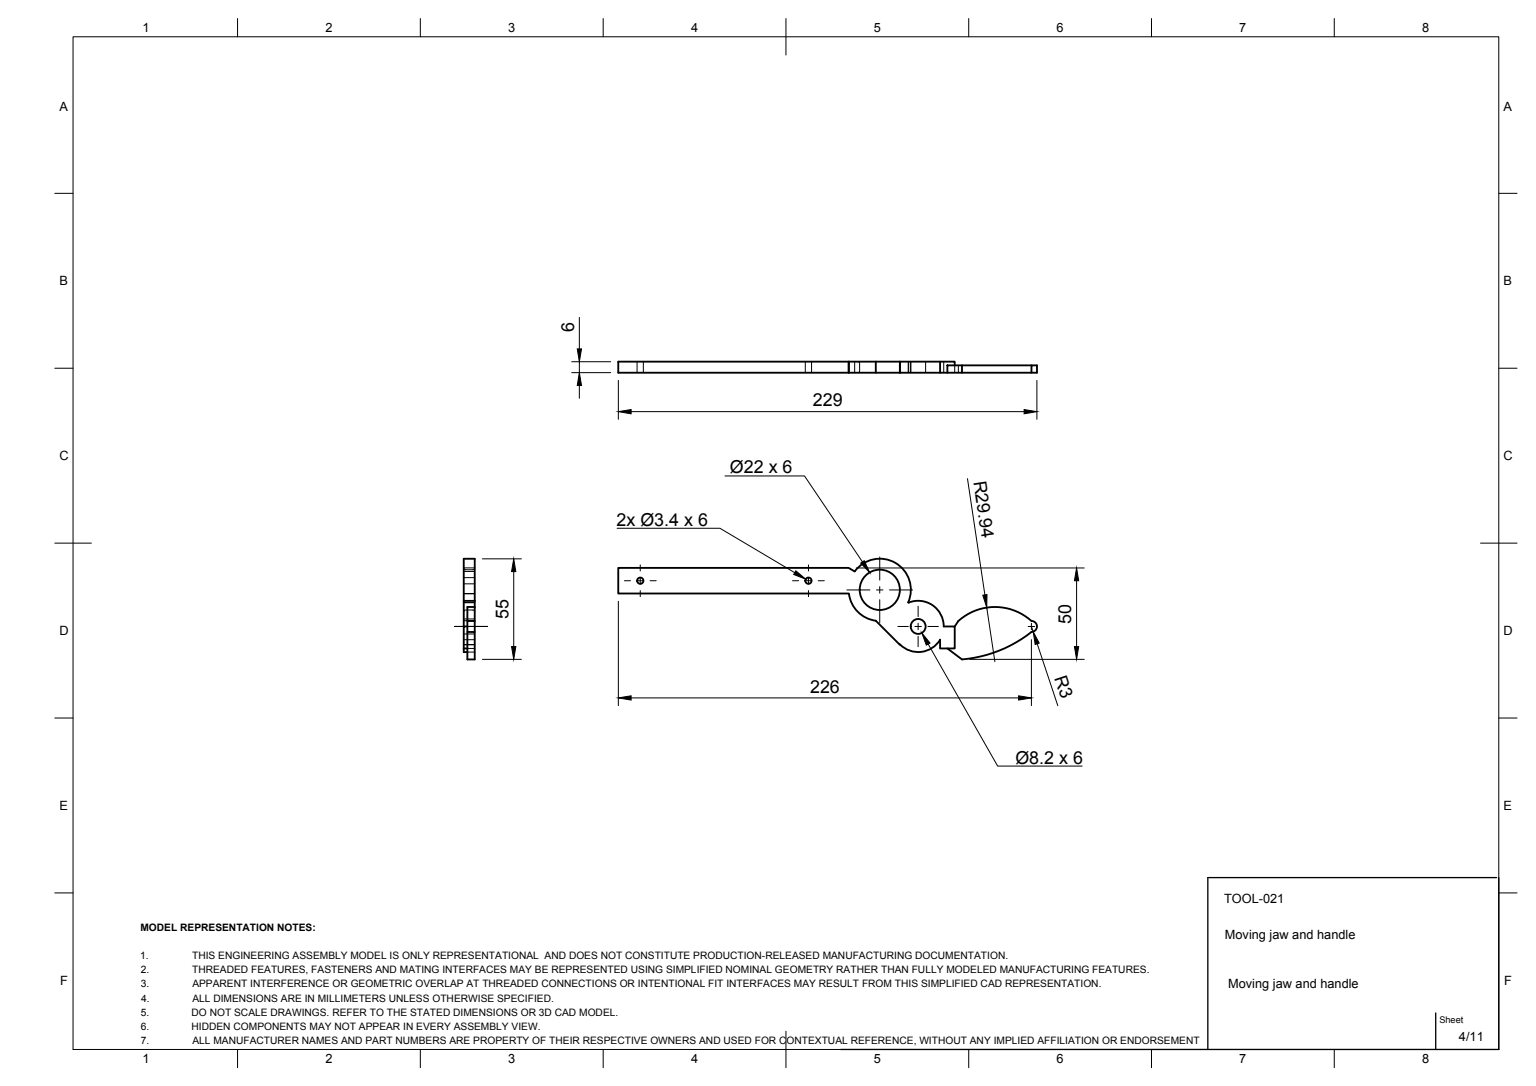
ISO-10303-21;
HEADER;
/* Generated by software containing ST-Developer
 * from STEP Tools, Inc. (www.steptools.com) 
 */

FILE_DESCRIPTION(
/* description */ (''),
/* implementation_level */ '2;1');

FILE_NAME(
/* name */ 'Moving jaw and handle.step',
/* time_stamp */ '2026-11-10T09:05:57-08:00',
/* author */ (''),
/* organization */ (''),
/* preprocessor_version */ 'ST-DEVELOPER v20.2',
/* originating_system */ 'Autodesk Translation Framework v15.17.0.0',
/* authorisation */ '');

FILE_SCHEMA (('AUTOMOTIVE_DESIGN { 1 0 10303 214 3 1 1 }'));
ENDSEC;

DATA;
#10=MECHANICAL_DESIGN_GEOMETRIC_PRESENTATION_REPRESENTATION('',(#566),#19618);
#546=SHAPE_REPRESENTATION_RELATIONSHIP('SRR','None',#19665,#556);
#556=ADVANCED_BREP_SHAPE_REPRESENTATION('',(#576),#19608);
#566=STYLED_ITEM('',(#19728),#576);
#576=MANIFOLD_SOLID_BREP('Body1',#7104);
#587=TOROIDAL_SURFACE('',#7321,1.2,0.1);
#588=TOROIDAL_SURFACE('',#7331,1.2,0.1);
#597=FACE_BOUND('',#1280,.T.);
#598=FACE_BOUND('',#1281,.T.);
#599=FACE_BOUND('',#1282,.T.);
#600=FACE_BOUND('',#1283,.T.);
#601=FACE_BOUND('',#1287,.T.);
#602=FACE_BOUND('',#1288,.T.);
#603=FACE_BOUND('',#1289,.T.);
#604=FACE_BOUND('',#1290,.T.);
#681=PLANE('',#7295);
#682=PLANE('',#7296);
#683=PLANE('',#7306);
#684=PLANE('',#7307);
#685=PLANE('',#7308);
#686=PLANE('',#7309);
#687=PLANE('',#7310);
#688=PLANE('',#7317);
#689=PLANE('',#7328);
#690=PLANE('',#7335);
#691=PLANE('',#7336);
#692=PLANE('',#7337);
#693=PLANE('',#7338);
#694=PLANE('',#7339);
#695=PLANE('',#7340);
#696=PLANE('',#7341);
#697=PLANE('',#7342);
#853=FACE_OUTER_BOUND('',#1264,.T.);
#854=FACE_OUTER_BOUND('',#1265,.T.);
#855=FACE_OUTER_BOUND('',#1266,.T.);
#856=FACE_OUTER_BOUND('',#1267,.T.);
#857=FACE_OUTER_BOUND('',#1268,.T.);
#858=FACE_OUTER_BOUND('',#1269,.T.);
#859=FACE_OUTER_BOUND('',#1270,.T.);
#860=FACE_OUTER_BOUND('',#1271,.T.);
#861=FACE_OUTER_BOUND('',#1272,.T.);
#862=FACE_OUTER_BOUND('',#1273,.T.);
#863=FACE_OUTER_BOUND('',#1274,.T.);
#864=FACE_OUTER_BOUND('',#1275,.T.);
#865=FACE_OUTER_BOUND('',#1276,.T.);
#866=FACE_OUTER_BOUND('',#1277,.T.);
#867=FACE_OUTER_BOUND('',#1278,.T.);
#868=FACE_OUTER_BOUND('',#1279,.T.);
#869=FACE_OUTER_BOUND('',#1284,.T.);
#870=FACE_OUTER_BOUND('',#1285,.T.);
#871=FACE_OUTER_BOUND('',#1286,.T.);
#872=FACE_OUTER_BOUND('',#1291,.T.);
#873=FACE_OUTER_BOUND('',#1292,.T.);
#874=FACE_OUTER_BOUND('',#1293,.T.);
#875=FACE_OUTER_BOUND('',#1294,.T.);
#876=FACE_OUTER_BOUND('',#1295,.T.);
#877=FACE_OUTER_BOUND('',#1296,.T.);
#878=FACE_OUTER_BOUND('',#1297,.T.);
#879=FACE_OUTER_BOUND('',#1298,.T.);
#880=FACE_OUTER_BOUND('',#1299,.T.);
#881=FACE_OUTER_BOUND('',#1300,.T.);
#882=FACE_OUTER_BOUND('',#1301,.T.);
#1264=EDGE_LOOP('',(#4678,#4679,#4680,#4681));
#1265=EDGE_LOOP('',(#4682,#4683,#4684,#4685));
#1266=EDGE_LOOP('',(#4686,#4687,#4688,#4689));
#1267=EDGE_LOOP('',(#4690,#4691,#4692,#4693));
#1268=EDGE_LOOP('',(#4694,#4695,#4696,#4697));
#1269=EDGE_LOOP('',(#4698,#4699,#4700,#4701));
#1270=EDGE_LOOP('',(#4702,#4703,#4704,#4705));
#1271=EDGE_LOOP('',(#4706,#4707,#4708,#4709));
#1272=EDGE_LOOP('',(#4710,#4711,#4712,#4713,#4714,#4715,#4716));
#1273=EDGE_LOOP('',(#4717,#4718,#4719,#4720,#4721,#4722));
#1274=EDGE_LOOP('',(#4723,#4724,#4725,#4726));
#1275=EDGE_LOOP('',(#4727,#4728,#4729,#4730,#4731));
#1276=EDGE_LOOP('',(#4732,#4733,#4734,#4735));
#1277=EDGE_LOOP('',(#4736,#4737,#4738,#4739));
#1278=EDGE_LOOP('',(#4740,#4741,#4742,#4743));
#1279=EDGE_LOOP('',(#4744,#4745,#4746,#4747,#4748,#4749,#4750,#4751,#4752,
#4753,#4754,#4755,#4756,#4757,#4758,#4759));
#1280=EDGE_LOOP('',(#4760));
#1281=EDGE_LOOP('',(#4761));
#1282=EDGE_LOOP('',(#4762));
#1283=EDGE_LOOP('',(#4763));
#1284=EDGE_LOOP('',(#4764,#4765,#4766,#4767));
#1285=EDGE_LOOP('',(#4768,#4769,#4770,#4771,#4772));
#1286=EDGE_LOOP('',(#4773,#4774,#4775,#4776,#4777,#4778,#4779,#4780,#4781,
#4782,#4783,#4784,#4785,#4786,#4787,#4788,#4789,#4790,#4791,#4792));
#1287=EDGE_LOOP('',(#4793));
#1288=EDGE_LOOP('',(#4794));
#1289=EDGE_LOOP('',(#4795));
#1290=EDGE_LOOP('',(#4796));
#1291=EDGE_LOOP('',(#4797,#4798,#4799,#4800,#4801));
#1292=EDGE_LOOP('',(#4802,#4803,#4804,#4805));
#1293=EDGE_LOOP('',(#4806,#4807,#4808,#4809));
#1294=EDGE_LOOP('',(#4810,#4811,#4812,#4813));
#1295=EDGE_LOOP('',(#4814,#4815,#4816,#4817));
#1296=EDGE_LOOP('',(#4818,#4819,#4820,#4821));
#1297=EDGE_LOOP('',(#4822,#4823,#4824,#4825));
#1298=EDGE_LOOP('',(#4826,#4827,#4828,#4829));
#1299=EDGE_LOOP('',(#4830,#4831,#4832,#4833));
#1300=EDGE_LOOP('',(#4834,#4835,#4836,#4837));
#1301=EDGE_LOOP('',(#4838,#4839,#4840,#4841));
#1758=LINE('',#9501,#2217);
#1759=LINE('',#9507,#2218);
#1760=LINE('',#9513,#2219);
#1761=LINE('',#9518,#2220);
#1762=LINE('',#9520,#2221);
#1763=LINE('',#9522,#2222);
#1764=LINE('',#9523,#2223);
#1765=LINE('',#9527,#2224);
#1766=LINE('',#9529,#2225);
#1767=LINE('',#9531,#2226);
#1768=LINE('',#9532,#2227);
#1769=LINE('',#9538,#2228);
#1770=LINE('',#9544,#2229);
#1771=LINE('',#9550,#2230);
#1772=LINE('',#9551,#2231);
#1773=LINE('',#9554,#2232);
#1774=LINE('',#9556,#2233);
#1775=LINE('',#9558,#2234);
#1776=LINE('',#9559,#2235);
#1777=LINE('',#9562,#2236);
#1778=LINE('',#9563,#2237);
#1779=LINE('',#9567,#2238);
#1780=LINE('',#9568,#2239);
#1781=LINE('',#9569,#2240);
#1782=LINE('',#9573,#2241);
#1783=LINE('',#9574,#2242);
#1784=LINE('',#9575,#2243);
#1785=LINE('',#9580,#2244);
#1786=LINE('',#9586,#2245);
#1787=LINE('',#9590,#2246);
#1788=LINE('',#9594,#2247);
#1789=LINE('',#9596,#2248);
#1790=LINE('',#9598,#2249);
#1791=LINE('',#9600,#2250);
#1792=LINE('',#9602,#2251);
#1793=LINE('',#9606,#2252);
#1794=LINE('',#9607,#2253);
#1795=LINE('',#9621,#2254);
#1796=LINE('',#9624,#2255);
#1797=LINE('',#9626,#2256);
#1798=LINE('',#9630,#2257);
#1799=LINE('',#9632,#2258);
#1800=LINE('',#9634,#2259);
#1801=LINE('',#9636,#2260);
#1802=LINE('',#9638,#2261);
#1803=LINE('',#9641,#2262);
#1804=LINE('',#9645,#2263);
#1805=LINE('',#9646,#2264);
#1806=LINE('',#9648,#2265);
#1807=LINE('',#9649,#2266);
#1808=LINE('',#9651,#2267);
#1809=LINE('',#9653,#2268);
#1810=LINE('',#9656,#2269);
#1811=LINE('',#9659,#2270);
#1812=LINE('',#9661,#2271);
#2217=VECTOR('',#7957,0.17);
#2218=VECTOR('',#7964,0.17);
#2219=VECTOR('',#7971,0.41);
#2220=VECTOR('',#7976,1.);
#2221=VECTOR('',#7977,1.);
#2222=VECTOR('',#7978,1.);
#2223=VECTOR('',#7979,1.);
#2224=VECTOR('',#7982,1.);
#2225=VECTOR('',#7983,1.);
#2226=VECTOR('',#7984,1.);
#2227=VECTOR('',#7985,1.);
#2228=VECTOR('',#7992,1.);
#2229=VECTOR('',#7999,1.);
#2230=VECTOR('',#8008,1.);
#2231=VECTOR('',#8009,1.);
#2232=VECTOR('',#8012,1.);
#2233=VECTOR('',#8013,1.);
#2234=VECTOR('',#8014,1.);
#2235=VECTOR('',#8015,1.);
#2236=VECTOR('',#8018,1.);
#2237=VECTOR('',#8019,1.);
#2238=VECTOR('',#8022,1.);
#2239=VECTOR('',#8023,1.);
#2240=VECTOR('',#8024,1.);
#2241=VECTOR('',#8027,1.);
#2242=VECTOR('',#8028,1.);
#2243=VECTOR('',#8029,1.);
#2244=VECTOR('',#8034,1.);
#2245=VECTOR('',#8041,1.);
#2246=VECTOR('',#8046,1.);
#2247=VECTOR('',#8049,1.);
#2248=VECTOR('',#8050,1.);
#2249=VECTOR('',#8051,1.);
#2250=VECTOR('',#8052,1.);
#2251=VECTOR('',#8053,1.);
#2252=VECTOR('',#8056,1.);
#2253=VECTOR('',#8057,1.);
#2254=VECTOR('',#8074,1.1);
#2255=VECTOR('',#8077,1.);
#2256=VECTOR('',#8078,1.);
#2257=VECTOR('',#8081,1.);
#2258=VECTOR('',#8082,1.);
#2259=VECTOR('',#8083,1.);
#2260=VECTOR('',#8084,1.);
#2261=VECTOR('',#8085,1.);
#2262=VECTOR('',#8088,1.);
#2263=VECTOR('',#8095,1.);
#2264=VECTOR('',#8096,1.);
#2265=VECTOR('',#8099,1.);
#2266=VECTOR('',#8100,1.);
#2267=VECTOR('',#8103,1.);
#2268=VECTOR('',#8106,1.);
#2269=VECTOR('',#8111,1.);
#2270=VECTOR('',#8116,1.);
#2271=VECTOR('',#8119,1.);
#2643=CIRCLE('',#7287,0.17);
#2644=CIRCLE('',#7288,0.17);
#2645=CIRCLE('',#7290,0.17);
#2646=CIRCLE('',#7291,0.17);
#2647=CIRCLE('',#7293,0.41);
#2648=CIRCLE('',#7294,0.41);
#2649=CIRCLE('',#7298,2.9940843367589);
#2650=CIRCLE('',#7299,2.9940843367589);
#2651=CIRCLE('',#7301,0.3);
#2652=CIRCLE('',#7302,0.3);
#2653=CIRCLE('',#7304,7.11398555645532);
#2654=CIRCLE('',#7305,7.11398555645532);
#2655=CIRCLE('',#7312,1.4);
#2656=CIRCLE('',#7313,1.4);
#2657=CIRCLE('',#7315,1.4);
#2658=CIRCLE('',#7316,1.4);
#2659=CIRCLE('',#7318,1.7);
#2660=CIRCLE('',#7319,1.7);
#2661=CIRCLE('',#7320,1.2);
#2662=CIRCLE('',#7322,1.2);
#2663=CIRCLE('',#7323,0.1);
#2664=CIRCLE('',#7324,1.1);
#2665=CIRCLE('',#7326,1.1);
#2666=CIRCLE('',#7327,1.1);
#2667=CIRCLE('',#7329,1.7);
#2668=CIRCLE('',#7330,1.7);
#2669=CIRCLE('',#7332,0.1);
#2867=VERTEX_POINT('',#9498);
#2868=VERTEX_POINT('',#9500);
#2869=VERTEX_POINT('',#9504);
#2870=VERTEX_POINT('',#9506);
#2871=VERTEX_POINT('',#9510);
#2872=VERTEX_POINT('',#9512);
#2873=VERTEX_POINT('',#9516);
#2874=VERTEX_POINT('',#9517);
#2875=VERTEX_POINT('',#9519);
#2876=VERTEX_POINT('',#9521);
#2877=VERTEX_POINT('',#9525);
#2878=VERTEX_POINT('',#9526);
#2879=VERTEX_POINT('',#9528);
#2880=VERTEX_POINT('',#9530);
#2881=VERTEX_POINT('',#9534);
#2882=VERTEX_POINT('',#9536);
#2883=VERTEX_POINT('',#9540);
#2884=VERTEX_POINT('',#9542);
#2885=VERTEX_POINT('',#9549);
#2886=VERTEX_POINT('',#9553);
#2887=VERTEX_POINT('',#9555);
#2888=VERTEX_POINT('',#9557);
#2889=VERTEX_POINT('',#9561);
#2890=VERTEX_POINT('',#9565);
#2891=VERTEX_POINT('',#9566);
#2892=VERTEX_POINT('',#9571);
#2893=VERTEX_POINT('',#9572);
#2894=VERTEX_POINT('',#9577);
#2895=VERTEX_POINT('',#9579);
#2896=VERTEX_POINT('',#9583);
#2897=VERTEX_POINT('',#9585);
#2898=VERTEX_POINT('',#9589);
#2899=VERTEX_POINT('',#9591);
#2900=VERTEX_POINT('',#9593);
#2901=VERTEX_POINT('',#9595);
#2902=VERTEX_POINT('',#9597);
#2903=VERTEX_POINT('',#9599);
#2904=VERTEX_POINT('',#9601);
#2905=VERTEX_POINT('',#9603);
#2906=VERTEX_POINT('',#9605);
#2907=VERTEX_POINT('',#9608);
#2908=VERTEX_POINT('',#9611);
#2909=VERTEX_POINT('',#9613);
#2910=VERTEX_POINT('',#9617);
#2911=VERTEX_POINT('',#9618);
#2912=VERTEX_POINT('',#9623);
#2913=VERTEX_POINT('',#9625);
#2914=VERTEX_POINT('',#9627);
#2915=VERTEX_POINT('',#9629);
#2916=VERTEX_POINT('',#9631);
#2917=VERTEX_POINT('',#9633);
#2918=VERTEX_POINT('',#9635);
#2919=VERTEX_POINT('',#9637);
#2920=VERTEX_POINT('',#9639);
#3564=EDGE_CURVE('',#2867,#2867,#2643,.T.);
#3565=EDGE_CURVE('',#2867,#2868,#1758,.T.);
#3566=EDGE_CURVE('',#2868,#2868,#2644,.T.);
#3567=EDGE_CURVE('',#2869,#2869,#2645,.T.);
#3568=EDGE_CURVE('',#2869,#2870,#1759,.T.);
#3569=EDGE_CURVE('',#2870,#2870,#2646,.T.);
#3570=EDGE_CURVE('',#2871,#2871,#2647,.T.);
#3571=EDGE_CURVE('',#2871,#2872,#1760,.T.);
#3572=EDGE_CURVE('',#2872,#2872,#2648,.T.);
#3573=EDGE_CURVE('',#2873,#2874,#1761,.T.);
#3574=EDGE_CURVE('',#2875,#2874,#1762,.T.);
#3575=EDGE_CURVE('',#2876,#2875,#1763,.T.);
#3576=EDGE_CURVE('',#2873,#2876,#1764,.T.);
#3577=EDGE_CURVE('',#2877,#2878,#1765,.T.);
#3578=EDGE_CURVE('',#2877,#2879,#1766,.T.);
#3579=EDGE_CURVE('',#2880,#2879,#1767,.T.);
#3580=EDGE_CURVE('',#2878,#2880,#1768,.T.);
#3581=EDGE_CURVE('',#2881,#2876,#2649,.T.);
#3582=EDGE_CURVE('',#2882,#2875,#2650,.T.);
#3583=EDGE_CURVE('',#2881,#2882,#1769,.T.);
#3584=EDGE_CURVE('',#2883,#2881,#2651,.T.);
#3585=EDGE_CURVE('',#2884,#2882,#2652,.T.);
#3586=EDGE_CURVE('',#2883,#2884,#1770,.T.);
#3587=EDGE_CURVE('',#2877,#2883,#2653,.T.);
#3588=EDGE_CURVE('',#2879,#2884,#2654,.T.);
#3589=EDGE_CURVE('',#2880,#2885,#1771,.T.);
#3590=EDGE_CURVE('',#2885,#2874,#1772,.T.);
#3591=EDGE_CURVE('',#2885,#2886,#1773,.T.);
#3592=EDGE_CURVE('',#2887,#2886,#1774,.T.);
#3593=EDGE_CURVE('',#2888,#2887,#1775,.T.);
#3594=EDGE_CURVE('',#2878,#2888,#1776,.T.);
#3595=EDGE_CURVE('',#2874,#2889,#1777,.T.);
#3596=EDGE_CURVE('',#2886,#2889,#1778,.T.);
#3597=EDGE_CURVE('',#2890,#2891,#1779,.T.);
#3598=EDGE_CURVE('',#2889,#2890,#1780,.T.);
#3599=EDGE_CURVE('',#2891,#2873,#1781,.T.);
#3600=EDGE_CURVE('',#2892,#2893,#1782,.T.);
#3601=EDGE_CURVE('',#2888,#2892,#1783,.T.);
#3602=EDGE_CURVE('',#2893,#2887,#1784,.T.);
#3603=EDGE_CURVE('',#2891,#2894,#2655,.T.);
#3604=EDGE_CURVE('',#2894,#2895,#1785,.T.);
#3605=EDGE_CURVE('',#2890,#2895,#2656,.T.);
#3606=EDGE_CURVE('',#2896,#2893,#2657,.T.);
#3607=EDGE_CURVE('',#2896,#2897,#1786,.T.);
#3608=EDGE_CURVE('',#2897,#2892,#2658,.T.);
#3609=EDGE_CURVE('',#2895,#2898,#1787,.T.);
#3610=EDGE_CURVE('',#2898,#2899,#2659,.T.);
#3611=EDGE_CURVE('',#2899,#2900,#1788,.T.);
#3612=EDGE_CURVE('',#2900,#2901,#1789,.T.);
#3613=EDGE_CURVE('',#2901,#2902,#1790,.T.);
#3614=EDGE_CURVE('',#2902,#2903,#1791,.T.);
#3615=EDGE_CURVE('',#2903,#2904,#1792,.T.);
#3616=EDGE_CURVE('',#2904,#2905,#2660,.T.);
#3617=EDGE_CURVE('',#2905,#2906,#1793,.T.);
#3618=EDGE_CURVE('',#2906,#2896,#1794,.T.);
#3619=EDGE_CURVE('',#2907,#2907,#2661,.T.);
#3620=EDGE_CURVE('',#2908,#2908,#2662,.T.);
#3621=EDGE_CURVE('',#2908,#2909,#2663,.T.);
#3622=EDGE_CURVE('',#2909,#2909,#2664,.T.);
#3623=EDGE_CURVE('',#2910,#2911,#2665,.T.);
#3624=EDGE_CURVE('',#2911,#2910,#2666,.T.);
#3625=EDGE_CURVE('',#2911,#2909,#1795,.T.);
#3626=EDGE_CURVE('',#2912,#2897,#1796,.T.);
#3627=EDGE_CURVE('',#2913,#2912,#1797,.T.);
#3628=EDGE_CURVE('',#2914,#2913,#2667,.T.);
#3629=EDGE_CURVE('',#2915,#2914,#1798,.T.);
#3630=EDGE_CURVE('',#2916,#2915,#1799,.T.);
#3631=EDGE_CURVE('',#2917,#2916,#1800,.T.);
#3632=EDGE_CURVE('',#2918,#2917,#1801,.T.);
#3633=EDGE_CURVE('',#2919,#2918,#1802,.T.);
#3634=EDGE_CURVE('',#2920,#2919,#2668,.T.);
#3635=EDGE_CURVE('',#2894,#2920,#1803,.T.);
#3636=EDGE_CURVE('',#2907,#2910,#2669,.T.);
#3637=EDGE_CURVE('',#2905,#2913,#1804,.T.);
#3638=EDGE_CURVE('',#2914,#2904,#1805,.T.);
#3639=EDGE_CURVE('',#2920,#2898,#1806,.T.);
#3640=EDGE_CURVE('',#2899,#2919,#1807,.T.);
#3641=EDGE_CURVE('',#2918,#2900,#1808,.T.);
#3642=EDGE_CURVE('',#2915,#2903,#1809,.T.);
#3643=EDGE_CURVE('',#2912,#2906,#1810,.T.);
#3644=EDGE_CURVE('',#2916,#2902,#1811,.T.);
#3645=EDGE_CURVE('',#2917,#2901,#1812,.T.);
#4678=ORIENTED_EDGE('',*,*,#3564,.F.);
#4679=ORIENTED_EDGE('',*,*,#3565,.T.);
#4680=ORIENTED_EDGE('',*,*,#3566,.F.);
#4681=ORIENTED_EDGE('',*,*,#3565,.F.);
#4682=ORIENTED_EDGE('',*,*,#3567,.F.);
#4683=ORIENTED_EDGE('',*,*,#3568,.T.);
#4684=ORIENTED_EDGE('',*,*,#3569,.F.);
#4685=ORIENTED_EDGE('',*,*,#3568,.F.);
#4686=ORIENTED_EDGE('',*,*,#3570,.F.);
#4687=ORIENTED_EDGE('',*,*,#3571,.T.);
#4688=ORIENTED_EDGE('',*,*,#3572,.F.);
#4689=ORIENTED_EDGE('',*,*,#3571,.F.);
#4690=ORIENTED_EDGE('',*,*,#3573,.T.);
#4691=ORIENTED_EDGE('',*,*,#3574,.F.);
#4692=ORIENTED_EDGE('',*,*,#3575,.F.);
#4693=ORIENTED_EDGE('',*,*,#3576,.F.);
#4694=ORIENTED_EDGE('',*,*,#3577,.F.);
#4695=ORIENTED_EDGE('',*,*,#3578,.T.);
#4696=ORIENTED_EDGE('',*,*,#3579,.F.);
#4697=ORIENTED_EDGE('',*,*,#3580,.F.);
#4698=ORIENTED_EDGE('',*,*,#3581,.T.);
#4699=ORIENTED_EDGE('',*,*,#3575,.T.);
#4700=ORIENTED_EDGE('',*,*,#3582,.F.);
#4701=ORIENTED_EDGE('',*,*,#3583,.F.);
#4702=ORIENTED_EDGE('',*,*,#3584,.T.);
#4703=ORIENTED_EDGE('',*,*,#3583,.T.);
#4704=ORIENTED_EDGE('',*,*,#3585,.F.);
#4705=ORIENTED_EDGE('',*,*,#3586,.F.);
#4706=ORIENTED_EDGE('',*,*,#3587,.T.);
#4707=ORIENTED_EDGE('',*,*,#3586,.T.);
#4708=ORIENTED_EDGE('',*,*,#3588,.F.);
#4709=ORIENTED_EDGE('',*,*,#3578,.F.);
#4710=ORIENTED_EDGE('',*,*,#3589,.F.);
#4711=ORIENTED_EDGE('',*,*,#3579,.T.);
#4712=ORIENTED_EDGE('',*,*,#3588,.T.);
#4713=ORIENTED_EDGE('',*,*,#3585,.T.);
#4714=ORIENTED_EDGE('',*,*,#3582,.T.);
#4715=ORIENTED_EDGE('',*,*,#3574,.T.);
#4716=ORIENTED_EDGE('',*,*,#3590,.F.);
#4717=ORIENTED_EDGE('',*,*,#3580,.T.);
#4718=ORIENTED_EDGE('',*,*,#3589,.T.);
#4719=ORIENTED_EDGE('',*,*,#3591,.T.);
#4720=ORIENTED_EDGE('',*,*,#3592,.F.);
#4721=ORIENTED_EDGE('',*,*,#3593,.F.);
#4722=ORIENTED_EDGE('',*,*,#3594,.F.);
#4723=ORIENTED_EDGE('',*,*,#3590,.T.);
#4724=ORIENTED_EDGE('',*,*,#3595,.T.);
#4725=ORIENTED_EDGE('',*,*,#3596,.F.);
#4726=ORIENTED_EDGE('',*,*,#3591,.F.);
#4727=ORIENTED_EDGE('',*,*,#3597,.F.);
#4728=ORIENTED_EDGE('',*,*,#3598,.F.);
#4729=ORIENTED_EDGE('',*,*,#3595,.F.);
#4730=ORIENTED_EDGE('',*,*,#3573,.F.);
#4731=ORIENTED_EDGE('',*,*,#3599,.F.);
#4732=ORIENTED_EDGE('',*,*,#3600,.F.);
#4733=ORIENTED_EDGE('',*,*,#3601,.F.);
#4734=ORIENTED_EDGE('',*,*,#3593,.T.);
#4735=ORIENTED_EDGE('',*,*,#3602,.F.);
#4736=ORIENTED_EDGE('',*,*,#3597,.T.);
#4737=ORIENTED_EDGE('',*,*,#3603,.T.);
#4738=ORIENTED_EDGE('',*,*,#3604,.T.);
#4739=ORIENTED_EDGE('',*,*,#3605,.F.);
#4740=ORIENTED_EDGE('',*,*,#3600,.T.);
#4741=ORIENTED_EDGE('',*,*,#3606,.F.);
#4742=ORIENTED_EDGE('',*,*,#3607,.T.);
#4743=ORIENTED_EDGE('',*,*,#3608,.T.);
#4744=ORIENTED_EDGE('',*,*,#3605,.T.);
#4745=ORIENTED_EDGE('',*,*,#3609,.T.);
#4746=ORIENTED_EDGE('',*,*,#3610,.T.);
#4747=ORIENTED_EDGE('',*,*,#3611,.T.);
#4748=ORIENTED_EDGE('',*,*,#3612,.T.);
#4749=ORIENTED_EDGE('',*,*,#3613,.T.);
#4750=ORIENTED_EDGE('',*,*,#3614,.T.);
#4751=ORIENTED_EDGE('',*,*,#3615,.T.);
#4752=ORIENTED_EDGE('',*,*,#3616,.T.);
#4753=ORIENTED_EDGE('',*,*,#3617,.T.);
#4754=ORIENTED_EDGE('',*,*,#3618,.T.);
#4755=ORIENTED_EDGE('',*,*,#3606,.T.);
#4756=ORIENTED_EDGE('',*,*,#3602,.T.);
#4757=ORIENTED_EDGE('',*,*,#3592,.T.);
#4758=ORIENTED_EDGE('',*,*,#3596,.T.);
#4759=ORIENTED_EDGE('',*,*,#3598,.T.);
#4760=ORIENTED_EDGE('',*,*,#3564,.T.);
#4761=ORIENTED_EDGE('',*,*,#3567,.T.);
#4762=ORIENTED_EDGE('',*,*,#3570,.T.);
#4763=ORIENTED_EDGE('',*,*,#3619,.F.);
#4764=ORIENTED_EDGE('',*,*,#3620,.T.);
#4765=ORIENTED_EDGE('',*,*,#3621,.T.);
#4766=ORIENTED_EDGE('',*,*,#3622,.T.);
#4767=ORIENTED_EDGE('',*,*,#3621,.F.);
#4768=ORIENTED_EDGE('',*,*,#3623,.F.);
#4769=ORIENTED_EDGE('',*,*,#3624,.F.);
#4770=ORIENTED_EDGE('',*,*,#3625,.T.);
#4771=ORIENTED_EDGE('',*,*,#3622,.F.);
#4772=ORIENTED_EDGE('',*,*,#3625,.F.);
#4773=ORIENTED_EDGE('',*,*,#3594,.T.);
#4774=ORIENTED_EDGE('',*,*,#3601,.T.);
#4775=ORIENTED_EDGE('',*,*,#3608,.F.);
#4776=ORIENTED_EDGE('',*,*,#3626,.F.);
#4777=ORIENTED_EDGE('',*,*,#3627,.F.);
#4778=ORIENTED_EDGE('',*,*,#3628,.F.);
#4779=ORIENTED_EDGE('',*,*,#3629,.F.);
#4780=ORIENTED_EDGE('',*,*,#3630,.F.);
#4781=ORIENTED_EDGE('',*,*,#3631,.F.);
#4782=ORIENTED_EDGE('',*,*,#3632,.F.);
#4783=ORIENTED_EDGE('',*,*,#3633,.F.);
#4784=ORIENTED_EDGE('',*,*,#3634,.F.);
#4785=ORIENTED_EDGE('',*,*,#3635,.F.);
#4786=ORIENTED_EDGE('',*,*,#3603,.F.);
#4787=ORIENTED_EDGE('',*,*,#3599,.T.);
#4788=ORIENTED_EDGE('',*,*,#3576,.T.);
#4789=ORIENTED_EDGE('',*,*,#3581,.F.);
#4790=ORIENTED_EDGE('',*,*,#3584,.F.);
#4791=ORIENTED_EDGE('',*,*,#3587,.F.);
#4792=ORIENTED_EDGE('',*,*,#3577,.T.);
#4793=ORIENTED_EDGE('',*,*,#3566,.T.);
#4794=ORIENTED_EDGE('',*,*,#3569,.T.);
#4795=ORIENTED_EDGE('',*,*,#3572,.T.);
#4796=ORIENTED_EDGE('',*,*,#3620,.F.);
#4797=ORIENTED_EDGE('',*,*,#3619,.T.);
#4798=ORIENTED_EDGE('',*,*,#3636,.T.);
#4799=ORIENTED_EDGE('',*,*,#3623,.T.);
#4800=ORIENTED_EDGE('',*,*,#3624,.T.);
#4801=ORIENTED_EDGE('',*,*,#3636,.F.);
#4802=ORIENTED_EDGE('',*,*,#3637,.F.);
#4803=ORIENTED_EDGE('',*,*,#3616,.F.);
#4804=ORIENTED_EDGE('',*,*,#3638,.F.);
#4805=ORIENTED_EDGE('',*,*,#3628,.T.);
#4806=ORIENTED_EDGE('',*,*,#3639,.F.);
#4807=ORIENTED_EDGE('',*,*,#3634,.T.);
#4808=ORIENTED_EDGE('',*,*,#3640,.F.);
#4809=ORIENTED_EDGE('',*,*,#3610,.F.);
#4810=ORIENTED_EDGE('',*,*,#3640,.T.);
#4811=ORIENTED_EDGE('',*,*,#3633,.T.);
#4812=ORIENTED_EDGE('',*,*,#3641,.T.);
#4813=ORIENTED_EDGE('',*,*,#3611,.F.);
#4814=ORIENTED_EDGE('',*,*,#3638,.T.);
#4815=ORIENTED_EDGE('',*,*,#3615,.F.);
#4816=ORIENTED_EDGE('',*,*,#3642,.F.);
#4817=ORIENTED_EDGE('',*,*,#3629,.T.);
#4818=ORIENTED_EDGE('',*,*,#3639,.T.);
#4819=ORIENTED_EDGE('',*,*,#3609,.F.);
#4820=ORIENTED_EDGE('',*,*,#3604,.F.);
#4821=ORIENTED_EDGE('',*,*,#3635,.T.);
#4822=ORIENTED_EDGE('',*,*,#3607,.F.);
#4823=ORIENTED_EDGE('',*,*,#3618,.F.);
#4824=ORIENTED_EDGE('',*,*,#3643,.F.);
#4825=ORIENTED_EDGE('',*,*,#3626,.T.);
#4826=ORIENTED_EDGE('',*,*,#3637,.T.);
#4827=ORIENTED_EDGE('',*,*,#3627,.T.);
#4828=ORIENTED_EDGE('',*,*,#3643,.T.);
#4829=ORIENTED_EDGE('',*,*,#3617,.F.);
#4830=ORIENTED_EDGE('',*,*,#3630,.T.);
#4831=ORIENTED_EDGE('',*,*,#3642,.T.);
#4832=ORIENTED_EDGE('',*,*,#3614,.F.);
#4833=ORIENTED_EDGE('',*,*,#3644,.F.);
#4834=ORIENTED_EDGE('',*,*,#3631,.T.);
#4835=ORIENTED_EDGE('',*,*,#3644,.T.);
#4836=ORIENTED_EDGE('',*,*,#3613,.F.);
#4837=ORIENTED_EDGE('',*,*,#3645,.F.);
#4838=ORIENTED_EDGE('',*,*,#3632,.T.);
#4839=ORIENTED_EDGE('',*,*,#3645,.T.);
#4840=ORIENTED_EDGE('',*,*,#3612,.F.);
#4841=ORIENTED_EDGE('',*,*,#3641,.F.);
#6568=CYLINDRICAL_SURFACE('',#7286,0.17);
#6569=CYLINDRICAL_SURFACE('',#7289,0.17);
#6570=CYLINDRICAL_SURFACE('',#7292,0.41);
#6571=CYLINDRICAL_SURFACE('',#7297,2.9940843367589);
#6572=CYLINDRICAL_SURFACE('',#7300,0.3);
#6573=CYLINDRICAL_SURFACE('',#7303,7.11398555645532);
#6574=CYLINDRICAL_SURFACE('',#7311,1.4);
#6575=CYLINDRICAL_SURFACE('',#7314,1.4);
#6576=CYLINDRICAL_SURFACE('',#7325,1.1);
#6577=CYLINDRICAL_SURFACE('',#7333,1.7);
#6578=CYLINDRICAL_SURFACE('',#7334,1.7);
#6732=ADVANCED_FACE('',(#853),#6568,.F.);
#6733=ADVANCED_FACE('',(#854),#6569,.F.);
#6734=ADVANCED_FACE('',(#855),#6570,.F.);
#6735=ADVANCED_FACE('',(#856),#681,.T.);
#6736=ADVANCED_FACE('',(#857),#682,.T.);
#6737=ADVANCED_FACE('',(#858),#6571,.T.);
#6738=ADVANCED_FACE('',(#859),#6572,.T.);
#6739=ADVANCED_FACE('',(#860),#6573,.T.);
#6740=ADVANCED_FACE('',(#861),#683,.T.);
#6741=ADVANCED_FACE('',(#862),#684,.T.);
#6742=ADVANCED_FACE('',(#863),#685,.T.);
#6743=ADVANCED_FACE('',(#864),#686,.T.);
#6744=ADVANCED_FACE('',(#865),#687,.T.);
#6745=ADVANCED_FACE('',(#866),#6574,.T.);
#6746=ADVANCED_FACE('',(#867),#6575,.T.);
#6747=ADVANCED_FACE('',(#868,#597,#598,#599,#600),#688,.T.);
#6748=ADVANCED_FACE('',(#869),#587,.T.);
#6749=ADVANCED_FACE('',(#870),#6576,.F.);
#6750=ADVANCED_FACE('',(#871,#601,#602,#603,#604),#689,.F.);
#6751=ADVANCED_FACE('',(#872),#588,.T.);
#6752=ADVANCED_FACE('',(#873),#6577,.T.);
#6753=ADVANCED_FACE('',(#874),#6578,.T.);
#6754=ADVANCED_FACE('',(#875),#690,.T.);
#6755=ADVANCED_FACE('',(#876),#691,.T.);
#6756=ADVANCED_FACE('',(#877),#692,.T.);
#6757=ADVANCED_FACE('',(#878),#693,.T.);
#6758=ADVANCED_FACE('',(#879),#694,.T.);
#6759=ADVANCED_FACE('',(#880),#695,.T.);
#6760=ADVANCED_FACE('',(#881),#696,.T.);
#6761=ADVANCED_FACE('',(#882),#697,.T.);
#7104=CLOSED_SHELL('',(#6732,#6733,#6734,#6735,#6736,#6737,#6738,#6739,
#6740,#6741,#6742,#6743,#6744,#6745,#6746,#6747,#6748,#6749,#6750,#6751,
#6752,#6753,#6754,#6755,#6756,#6757,#6758,#6759,#6760,#6761));
#7285=AXIS2_PLACEMENT_3D('',#9496,#7951,#7952);
#7286=AXIS2_PLACEMENT_3D('',#9497,#7953,#7954);
#7287=AXIS2_PLACEMENT_3D('',#9499,#7955,#7956);
#7288=AXIS2_PLACEMENT_3D('',#9502,#7958,#7959);
#7289=AXIS2_PLACEMENT_3D('',#9503,#7960,#7961);
#7290=AXIS2_PLACEMENT_3D('',#9505,#7962,#7963);
#7291=AXIS2_PLACEMENT_3D('',#9508,#7965,#7966);
#7292=AXIS2_PLACEMENT_3D('',#9509,#7967,#7968);
#7293=AXIS2_PLACEMENT_3D('',#9511,#7969,#7970);
#7294=AXIS2_PLACEMENT_3D('',#9514,#7972,#7973);
#7295=AXIS2_PLACEMENT_3D('',#9515,#7974,#7975);
#7296=AXIS2_PLACEMENT_3D('',#9524,#7980,#7981);
#7297=AXIS2_PLACEMENT_3D('',#9533,#7986,#7987);
#7298=AXIS2_PLACEMENT_3D('',#9535,#7988,#7989);
#7299=AXIS2_PLACEMENT_3D('',#9537,#7990,#7991);
#7300=AXIS2_PLACEMENT_3D('',#9539,#7993,#7994);
#7301=AXIS2_PLACEMENT_3D('',#9541,#7995,#7996);
#7302=AXIS2_PLACEMENT_3D('',#9543,#7997,#7998);
#7303=AXIS2_PLACEMENT_3D('',#9545,#8000,#8001);
#7304=AXIS2_PLACEMENT_3D('',#9546,#8002,#8003);
#7305=AXIS2_PLACEMENT_3D('',#9547,#8004,#8005);
#7306=AXIS2_PLACEMENT_3D('',#9548,#8006,#8007);
#7307=AXIS2_PLACEMENT_3D('',#9552,#8010,#8011);
#7308=AXIS2_PLACEMENT_3D('',#9560,#8016,#8017);
#7309=AXIS2_PLACEMENT_3D('',#9564,#8020,#8021);
#7310=AXIS2_PLACEMENT_3D('',#9570,#8025,#8026);
#7311=AXIS2_PLACEMENT_3D('',#9576,#8030,#8031);
#7312=AXIS2_PLACEMENT_3D('',#9578,#8032,#8033);
#7313=AXIS2_PLACEMENT_3D('',#9581,#8035,#8036);
#7314=AXIS2_PLACEMENT_3D('',#9582,#8037,#8038);
#7315=AXIS2_PLACEMENT_3D('',#9584,#8039,#8040);
#7316=AXIS2_PLACEMENT_3D('',#9587,#8042,#8043);
#7317=AXIS2_PLACEMENT_3D('',#9588,#8044,#8045);
#7318=AXIS2_PLACEMENT_3D('',#9592,#8047,#8048);
#7319=AXIS2_PLACEMENT_3D('',#9604,#8054,#8055);
#7320=AXIS2_PLACEMENT_3D('',#9609,#8058,#8059);
#7321=AXIS2_PLACEMENT_3D('',#9610,#8060,#8061);
#7322=AXIS2_PLACEMENT_3D('',#9612,#8062,#8063);
#7323=AXIS2_PLACEMENT_3D('',#9614,#8064,#8065);
#7324=AXIS2_PLACEMENT_3D('',#9615,#8066,#8067);
#7325=AXIS2_PLACEMENT_3D('',#9616,#8068,#8069);
#7326=AXIS2_PLACEMENT_3D('',#9619,#8070,#8071);
#7327=AXIS2_PLACEMENT_3D('',#9620,#8072,#8073);
#7328=AXIS2_PLACEMENT_3D('',#9622,#8075,#8076);
#7329=AXIS2_PLACEMENT_3D('',#9628,#8079,#8080);
#7330=AXIS2_PLACEMENT_3D('',#9640,#8086,#8087);
#7331=AXIS2_PLACEMENT_3D('',#9642,#8089,#8090);
#7332=AXIS2_PLACEMENT_3D('',#9643,#8091,#8092);
#7333=AXIS2_PLACEMENT_3D('',#9644,#8093,#8094);
#7334=AXIS2_PLACEMENT_3D('',#9647,#8097,#8098);
#7335=AXIS2_PLACEMENT_3D('',#9650,#8101,#8102);
#7336=AXIS2_PLACEMENT_3D('',#9652,#8104,#8105);
#7337=AXIS2_PLACEMENT_3D('',#9654,#8107,#8108);
#7338=AXIS2_PLACEMENT_3D('',#9655,#8109,#8110);
#7339=AXIS2_PLACEMENT_3D('',#9657,#8112,#8113);
#7340=AXIS2_PLACEMENT_3D('',#9658,#8114,#8115);
#7341=AXIS2_PLACEMENT_3D('',#9660,#8117,#8118);
#7342=AXIS2_PLACEMENT_3D('',#9662,#8120,#8121);
#7951=DIRECTION('axis',(0.,0.,1.));
#7952=DIRECTION('refdir',(1.,0.,0.));
#7953=DIRECTION('center_axis',(0.,0.,-1.));
#7954=DIRECTION('ref_axis',(1.,0.,0.));
#7955=DIRECTION('center_axis',(0.,0.,-1.));
#7956=DIRECTION('ref_axis',(1.,0.,0.));
#7957=DIRECTION('',(0.,0.,-1.));
#7958=DIRECTION('center_axis',(0.,0.,1.));
#7959=DIRECTION('ref_axis',(1.,0.,0.));
#7960=DIRECTION('center_axis',(0.,0.,-1.));
#7961=DIRECTION('ref_axis',(1.,0.,0.));
#7962=DIRECTION('center_axis',(0.,0.,-1.));
#7963=DIRECTION('ref_axis',(1.,0.,0.));
#7964=DIRECTION('',(0.,0.,-1.));
#7965=DIRECTION('center_axis',(0.,0.,1.));
#7966=DIRECTION('ref_axis',(1.,0.,0.));
#7967=DIRECTION('center_axis',(0.,0.,-1.));
#7968=DIRECTION('ref_axis',(1.,0.,0.));
#7969=DIRECTION('center_axis',(0.,0.,-1.));
#7970=DIRECTION('ref_axis',(1.,0.,0.));
#7971=DIRECTION('',(0.,0.,-1.));
#7972=DIRECTION('center_axis',(0.,0.,1.));
#7973=DIRECTION('ref_axis',(1.,0.,0.));
#7974=DIRECTION('center_axis',(0.832050294337844,-0.554700196225229,0.));
#7975=DIRECTION('ref_axis',(0.554700196225229,0.832050294337844,0.));
#7976=DIRECTION('',(0.,0.,1.));
#7977=DIRECTION('',(0.554700196225229,0.832050294337844,0.));
#7978=DIRECTION('',(0.,0.,1.));
#7979=DIRECTION('',(-0.554700196225229,-0.832050294337844,0.));
#7980=DIRECTION('center_axis',(0.6,0.8,0.));
#7981=DIRECTION('ref_axis',(-0.8,0.6,0.));
#7982=DIRECTION('',(0.8,-0.6,0.));
#7983=DIRECTION('',(0.,0.,1.));
#7984=DIRECTION('',(-0.8,0.6,0.));
#7985=DIRECTION('',(0.,0.,1.));
#7986=DIRECTION('center_axis',(0.,0.,1.));
#7987=DIRECTION('ref_axis',(-0.667983855847227,-0.744175764404802,0.));
#7988=DIRECTION('center_axis',(0.,0.,1.));
#7989=DIRECTION('ref_axis',(-0.667983855847227,-0.744175764404802,0.));
#7990=DIRECTION('center_axis',(0.,0.,1.));
#7991=DIRECTION('ref_axis',(-0.667983855847227,-0.744175764404802,0.));
#7992=DIRECTION('',(0.,0.,1.));
#7993=DIRECTION('center_axis',(0.,0.,1.));
#7994=DIRECTION('ref_axis',(-2.96059473233375E-15,1.,0.));
#7995=DIRECTION('center_axis',(0.,0.,1.));
#7996=DIRECTION('ref_axis',(-2.96059473233375E-15,1.,0.));
#7997=DIRECTION('center_axis',(0.,0.,1.));
#7998=DIRECTION('ref_axis',(-2.96059473233375E-15,1.,0.));
#7999=DIRECTION('',(0.,0.,1.));
#8000=DIRECTION('center_axis',(0.,0.,1.));
#8001=DIRECTION('ref_axis',(-0.0846257248853095,0.99641280937553,0.));
#8002=DIRECTION('center_axis',(0.,0.,1.));
#8003=DIRECTION('ref_axis',(-0.0846257248853095,0.99641280937553,0.));
#8004=DIRECTION('center_axis',(0.,0.,1.));
#8005=DIRECTION('ref_axis',(-0.0846257248853095,0.99641280937553,0.));
#8006=DIRECTION('center_axis',(0.,0.,1.));
#8007=DIRECTION('ref_axis',(1.,0.,0.));
#8008=DIRECTION('',(-1.,0.,0.));
#8009=DIRECTION('',(0.,-1.,0.));
#8010=DIRECTION('center_axis',(0.,1.,0.));
#8011=DIRECTION('ref_axis',(-1.,0.,0.));
#8012=DIRECTION('',(0.,0.,1.));
#8013=DIRECTION('',(-1.,0.,0.));
#8014=DIRECTION('',(0.,0.,1.));
#8015=DIRECTION('',(1.,0.,0.));
#8016=DIRECTION('center_axis',(-1.,0.,0.));
#8017=DIRECTION('ref_axis',(0.,-1.,0.));
#8018=DIRECTION('',(0.,0.,1.));
#8019=DIRECTION('',(0.,-1.,0.));
#8020=DIRECTION('center_axis',(0.,-1.,0.));
#8021=DIRECTION('ref_axis',(1.,0.,0.));
#8022=DIRECTION('',(0.,0.,-1.));
#8023=DIRECTION('',(1.,0.,0.));
#8024=DIRECTION('',(-1.,0.,0.));
#8025=DIRECTION('center_axis',(1.,0.,0.));
#8026=DIRECTION('ref_axis',(0.,1.,0.));
#8027=DIRECTION('',(0.,0.,1.));
#8028=DIRECTION('',(0.,-1.,0.));
#8029=DIRECTION('',(0.,1.,0.));
#8030=DIRECTION('center_axis',(0.,0.,1.));
#8031=DIRECTION('ref_axis',(1.,0.,0.));
#8032=DIRECTION('center_axis',(0.,0.,1.));
#8033=DIRECTION('ref_axis',(1.,0.,0.));
#8034=DIRECTION('',(0.,0.,1.));
#8035=DIRECTION('center_axis',(0.,0.,1.));
#8036=DIRECTION('ref_axis',(1.,0.,0.));
#8037=DIRECTION('center_axis',(0.,0.,1.));
#8038=DIRECTION('ref_axis',(1.,0.,0.));
#8039=DIRECTION('center_axis',(0.,0.,1.));
#8040=DIRECTION('ref_axis',(1.,0.,0.));
#8041=DIRECTION('',(0.,0.,-1.));
#8042=DIRECTION('center_axis',(0.,0.,1.));
#8043=DIRECTION('ref_axis',(1.,0.,0.));
#8044=DIRECTION('center_axis',(0.,0.,1.));
#8045=DIRECTION('ref_axis',(1.,0.,0.));
#8046=DIRECTION('',(0.865426285481126,-0.501036270541705,0.));
#8047=DIRECTION('center_axis',(0.,0.,1.));
#8048=DIRECTION('ref_axis',(1.,0.,0.));
#8049=DIRECTION('',(0.865426285481126,-0.501036270541705,0.));
#8050=DIRECTION('',(1.,0.,0.));
#8051=DIRECTION('',(0.,1.,0.));
#8052=DIRECTION('',(-1.,0.,0.));
#8053=DIRECTION('',(-0.707106781186548,0.707106781186548,0.));
#8054=DIRECTION('center_axis',(0.,0.,1.));
#8055=DIRECTION('ref_axis',(1.,0.,0.));
#8056=DIRECTION('',(-0.707106781186548,0.707106781186548,0.));
#8057=DIRECTION('',(-0.447213595499958,-0.894427190999916,0.));
#8058=DIRECTION('center_axis',(0.,0.,1.));
#8059=DIRECTION('ref_axis',(-1.,0.,0.));
#8060=DIRECTION('center_axis',(0.,0.,1.));
#8061=DIRECTION('ref_axis',(1.,0.,0.));
#8062=DIRECTION('center_axis',(0.,0.,-1.));
#8063=DIRECTION('ref_axis',(-1.,2.01858731750028E-16,0.));
#8064=DIRECTION('center_axis',(0.,-1.,0.));
#8065=DIRECTION('ref_axis',(-1.,0.,0.));
#8066=DIRECTION('center_axis',(0.,0.,1.));
#8067=DIRECTION('ref_axis',(-1.,2.01858731750028E-16,0.));
#8068=DIRECTION('center_axis',(0.,0.,-1.));
#8069=DIRECTION('ref_axis',(1.,0.,0.));
#8070=DIRECTION('center_axis',(0.,0.,-1.));
#8071=DIRECTION('ref_axis',(-1.,0.,0.));
#8072=DIRECTION('center_axis',(0.,0.,-1.));
#8073=DIRECTION('ref_axis',(-1.,0.,0.));
#8074=DIRECTION('',(0.,0.,-1.));
#8075=DIRECTION('center_axis',(0.,0.,1.));
#8076=DIRECTION('ref_axis',(1.,0.,0.));
#8077=DIRECTION('',(-0.447213595499958,-0.894427190999916,0.));
#8078=DIRECTION('',(-0.707106781186548,0.707106781186548,0.));
#8079=DIRECTION('center_axis',(0.,0.,1.));
#8080=DIRECTION('ref_axis',(1.,0.,0.));
#8081=DIRECTION('',(-0.707106781186548,0.707106781186548,0.));
#8082=DIRECTION('',(-1.,0.,0.));
#8083=DIRECTION('',(0.,1.,0.));
#8084=DIRECTION('',(1.,0.,0.));
#8085=DIRECTION('',(0.865426285481126,-0.501036270541705,0.));
#8086=DIRECTION('center_axis',(0.,0.,1.));
#8087=DIRECTION('ref_axis',(1.,0.,0.));
#8088=DIRECTION('',(0.865426285481126,-0.501036270541705,0.));
#8089=DIRECTION('center_axis',(0.,0.,-1.));
#8090=DIRECTION('ref_axis',(-1.,0.,0.));
#8091=DIRECTION('center_axis',(0.,-1.,0.));
#8092=DIRECTION('ref_axis',(1.,0.,0.));
#8093=DIRECTION('center_axis',(0.,0.,1.));
#8094=DIRECTION('ref_axis',(1.,0.,0.));
#8095=DIRECTION('',(0.,0.,-1.));
#8096=DIRECTION('',(0.,0.,1.));
#8097=DIRECTION('center_axis',(0.,0.,1.));
#8098=DIRECTION('ref_axis',(-0.501036270541705,-0.865426285481126,0.));
#8099=DIRECTION('',(0.,0.,1.));
#8100=DIRECTION('',(0.,0.,-1.));
#8101=DIRECTION('center_axis',(-0.501036270541705,-0.865426285481126,0.));
#8102=DIRECTION('ref_axis',(0.865426285481126,-0.501036270541705,0.));
#8103=DIRECTION('',(0.,0.,1.));
#8104=DIRECTION('center_axis',(0.707106781186548,0.707106781186548,0.));
#8105=DIRECTION('ref_axis',(-0.707106781186548,0.707106781186548,0.));
#8106=DIRECTION('',(0.,0.,1.));
#8107=DIRECTION('center_axis',(-0.501036270541705,-0.865426285481126,0.));
#8108=DIRECTION('ref_axis',(0.865426285481126,-0.501036270541705,0.));
#8109=DIRECTION('center_axis',(-0.894427190999916,0.447213595499958,0.));
#8110=DIRECTION('ref_axis',(-0.447213595499958,-0.894427190999916,0.));
#8111=DIRECTION('',(0.,0.,1.));
#8112=DIRECTION('center_axis',(0.707106781186548,0.707106781186548,0.));
#8113=DIRECTION('ref_axis',(-0.707106781186548,0.707106781186548,0.));
#8114=DIRECTION('center_axis',(0.,1.,0.));
#8115=DIRECTION('ref_axis',(-1.,0.,0.));
#8116=DIRECTION('',(0.,0.,1.));
#8117=DIRECTION('center_axis',(1.,0.,0.));
#8118=DIRECTION('ref_axis',(0.,1.,0.));
#8119=DIRECTION('',(0.,0.,1.));
#8120=DIRECTION('center_axis',(0.,-1.,0.));
#8121=DIRECTION('ref_axis',(1.,0.,0.));
#9496=CARTESIAN_POINT('',(0.,0.,0.));
#9497=CARTESIAN_POINT('Origin',(6.,-2.5,0.3));
#9498=CARTESIAN_POINT('',(5.83,-2.5,0.6));
#9499=CARTESIAN_POINT('Origin',(6.,-2.5,0.6));
#9500=CARTESIAN_POINT('',(5.83,-2.5,0.));
#9501=CARTESIAN_POINT('',(5.83,-2.5,0.3));
#9502=CARTESIAN_POINT('Origin',(6.,-2.5,0.));
#9503=CARTESIAN_POINT('Origin',(15.2,-2.5,0.3));
#9504=CARTESIAN_POINT('',(15.03,-2.5,0.6));
#9505=CARTESIAN_POINT('Origin',(15.2,-2.5,0.6));
#9506=CARTESIAN_POINT('',(15.03,-2.5,0.));
#9507=CARTESIAN_POINT('',(15.03,-2.5,0.3));
#9508=CARTESIAN_POINT('Origin',(15.2,-2.5,0.));
#9509=CARTESIAN_POINT('Origin',(0.,0.,0.3));
#9510=CARTESIAN_POINT('',(-0.41,5.02105187650415E-17,0.6));
#9511=CARTESIAN_POINT('Origin',(0.,0.,0.6));
#9512=CARTESIAN_POINT('',(-0.41,5.02105187650415E-17,0.));
#9513=CARTESIAN_POINT('',(-0.41,5.02105187650415E-17,0.3));
#9514=CARTESIAN_POINT('Origin',(0.,0.,0.));
#9515=CARTESIAN_POINT('Origin',(-2.2,-0.3,0.));
#9516=CARTESIAN_POINT('',(-2.,0.,0.));
#9517=CARTESIAN_POINT('',(-2.,0.,0.4));
#9518=CARTESIAN_POINT('',(-2.,0.,0.));
#9519=CARTESIAN_POINT('',(-2.2,-0.3,0.4));
#9520=CARTESIAN_POINT('',(-1.6,0.6,0.4));
#9521=CARTESIAN_POINT('',(-2.2,-0.3,0.));
#9522=CARTESIAN_POINT('',(-2.2,-0.3,0.));
#9523=CARTESIAN_POINT('',(-1.6,0.6,0.));
#9524=CARTESIAN_POINT('Origin',(-1.6,1.2,0.));
#9525=CARTESIAN_POINT('',(-2.4,1.8,0.));
#9526=CARTESIAN_POINT('',(-1.6,1.2,0.));
#9527=CARTESIAN_POINT('',(-2.4,1.8,0.));
#9528=CARTESIAN_POINT('',(-2.4,1.8,0.4));
#9529=CARTESIAN_POINT('',(-2.4,1.8,0.));
#9530=CARTESIAN_POINT('',(-1.6,1.2,0.4));
#9531=CARTESIAN_POINT('',(-2.4,1.8,0.4));
#9532=CARTESIAN_POINT('',(-1.6,1.2,0.));
#9533=CARTESIAN_POINT('Origin',(-4.2,1.928125,0.));
#9534=CARTESIAN_POINT('',(-6.2,-0.3,0.));
#9535=CARTESIAN_POINT('Origin',(-4.2,1.928125,0.));
#9536=CARTESIAN_POINT('',(-6.2,-0.3,0.4));
#9537=CARTESIAN_POINT('Origin',(-4.2,1.928125,0.4));
#9538=CARTESIAN_POINT('',(-6.2,-0.3,0.));
#9539=CARTESIAN_POINT('Origin',(-6.2,2.77555756156289E-17,0.));
#9540=CARTESIAN_POINT('',(-6.2,0.300000000000001,0.));
#9541=CARTESIAN_POINT('Origin',(-6.2,2.77555756156289E-17,0.));
#9542=CARTESIAN_POINT('',(-6.2,0.3,0.4));
#9543=CARTESIAN_POINT('Origin',(-6.2,2.77555756156289E-17,0.4));
#9544=CARTESIAN_POINT('',(-6.2,0.300000000000001,0.));
#9545=CARTESIAN_POINT('Origin',(-1.79797381546135,-5.28846633416459,0.));
#9546=CARTESIAN_POINT('Origin',(-1.79797381546135,-5.28846633416459,0.));
#9547=CARTESIAN_POINT('Origin',(-1.79797381546135,-5.28846633416459,0.4));
#9548=CARTESIAN_POINT('Origin',(-4.05,0.367020331620548,0.4));
#9549=CARTESIAN_POINT('',(-2.,1.2,0.4));
#9550=CARTESIAN_POINT('',(-2.625,1.2,0.4));
#9551=CARTESIAN_POINT('',(-2.,0.783510165810274,0.4));
#9552=CARTESIAN_POINT('Origin',(-1.2,1.2,0.));
#9553=CARTESIAN_POINT('',(-2.,1.2,0.6));
#9554=CARTESIAN_POINT('',(-2.,1.2,0.));
#9555=CARTESIAN_POINT('',(-1.2,1.2,0.6));
#9556=CARTESIAN_POINT('',(-2.,1.2,0.6));
#9557=CARTESIAN_POINT('',(-1.2,1.2,0.));
#9558=CARTESIAN_POINT('',(-1.2,1.2,0.));
#9559=CARTESIAN_POINT('',(-2.,1.2,0.));
#9560=CARTESIAN_POINT('Origin',(-2.,1.2,0.));
#9561=CARTESIAN_POINT('',(-2.,0.,0.6));
#9562=CARTESIAN_POINT('',(-2.,0.,0.));
#9563=CARTESIAN_POINT('',(-2.,0.,0.6));
#9564=CARTESIAN_POINT('Origin',(-2.,0.,0.));
#9565=CARTESIAN_POINT('',(-1.4,0.,0.6));
#9566=CARTESIAN_POINT('',(-1.4,0.,0.));
#9567=CARTESIAN_POINT('',(-1.4,0.,0.));
#9568=CARTESIAN_POINT('',(-1.2,0.,0.6));
#9569=CARTESIAN_POINT('',(-1.2,0.,0.));
#9570=CARTESIAN_POINT('Origin',(-1.2,0.,0.));
#9571=CARTESIAN_POINT('',(-1.2,0.721110255092798,0.));
#9572=CARTESIAN_POINT('',(-1.2,0.721110255092798,0.6));
#9573=CARTESIAN_POINT('',(-1.2,0.721110255092798,0.));
#9574=CARTESIAN_POINT('',(-1.2,1.2,0.));
#9575=CARTESIAN_POINT('',(-1.2,1.2,0.6));
#9576=CARTESIAN_POINT('Origin',(0.,0.,0.));
#9577=CARTESIAN_POINT('',(0.518766934059614,-1.30033875129767,0.));
#9578=CARTESIAN_POINT('Origin',(0.,0.,0.));
#9579=CARTESIAN_POINT('',(0.518766934059614,-1.30033875129767,0.6));
#9580=CARTESIAN_POINT('',(0.518766934059614,-1.30033875129767,0.));
#9581=CARTESIAN_POINT('Origin',(0.,0.,0.6));
#9582=CARTESIAN_POINT('Origin',(0.,0.,0.));
#9583=CARTESIAN_POINT('',(0.993295878967653,0.986591757935306,0.6));
#9584=CARTESIAN_POINT('Origin',(0.,0.,0.6));
#9585=CARTESIAN_POINT('',(0.993295878967653,0.986591757935306,0.));
#9586=CARTESIAN_POINT('',(0.993295878967653,0.986591757935306,0.));
#9587=CARTESIAN_POINT('Origin',(0.,0.,0.));
#9588=CARTESIAN_POINT('Origin',(0.,0.,0.6));
#9589=CARTESIAN_POINT('',(0.544110909138566,-1.31501157897496,0.6));
#9590=CARTESIAN_POINT('',(0.,-1.,0.6));
#9591=CARTESIAN_POINT('',(3.46875216140085,-3.00822493554786,0.6));
#9592=CARTESIAN_POINT('Origin',(2.1,-2.,0.6));
#9593=CARTESIAN_POINT('',(3.8,-3.2,0.6));
#9594=CARTESIAN_POINT('',(0.,-1.,0.6));
#9595=CARTESIAN_POINT('',(16.4,-3.2,0.6));
#9596=CARTESIAN_POINT('',(3.8,-3.2,0.6));
#9597=CARTESIAN_POINT('',(16.4,-1.8,0.6));
#9598=CARTESIAN_POINT('',(16.4,-3.2,0.6));
#9599=CARTESIAN_POINT('',(3.8,-1.8,0.6));
#9600=CARTESIAN_POINT('',(16.4,-1.8,0.6));
#9601=CARTESIAN_POINT('',(3.78654599313281,-1.78654599313281,0.6));
#9602=CARTESIAN_POINT('',(3.8,-1.8,0.6));
#9603=CARTESIAN_POINT('',(2.31345400686719,-0.313454006867188,0.6));
#9604=CARTESIAN_POINT('Origin',(2.1,-2.,0.6));
#9605=CARTESIAN_POINT('',(1.,1.,0.6));
#9606=CARTESIAN_POINT('',(3.8,-1.8,0.6));
#9607=CARTESIAN_POINT('',(1.,1.,0.6));
#9608=CARTESIAN_POINT('',(3.3,-2.,0.6));
#9609=CARTESIAN_POINT('Origin',(2.1,-2.,0.6));
#9610=CARTESIAN_POINT('Origin',(2.1,-2.,0.1));
#9611=CARTESIAN_POINT('',(0.9,-2.,0.));
#9612=CARTESIAN_POINT('Origin',(2.1,-2.,0.));
#9613=CARTESIAN_POINT('',(1.,-2.,0.1));
#9614=CARTESIAN_POINT('Origin',(0.9,-2.,0.1));
#9615=CARTESIAN_POINT('Origin',(2.1,-2.,0.1));
#9616=CARTESIAN_POINT('Origin',(2.1,-2.,0.3));
#9617=CARTESIAN_POINT('',(3.2,-2.,0.5));
#9618=CARTESIAN_POINT('',(1.,-2.,0.5));
#9619=CARTESIAN_POINT('Origin',(2.1,-2.,0.5));
#9620=CARTESIAN_POINT('Origin',(2.1,-2.,0.5));
#9621=CARTESIAN_POINT('',(1.,-2.,0.3));
#9622=CARTESIAN_POINT('Origin',(0.,0.,0.));
#9623=CARTESIAN_POINT('',(1.,1.,0.));
#9624=CARTESIAN_POINT('',(1.,1.,0.));
#9625=CARTESIAN_POINT('',(2.31345400686719,-0.313454006867188,0.));
#9626=CARTESIAN_POINT('',(3.8,-1.8,0.));
#9627=CARTESIAN_POINT('',(3.78654599313281,-1.78654599313281,0.));
#9628=CARTESIAN_POINT('Origin',(2.1,-2.,0.));
#9629=CARTESIAN_POINT('',(3.8,-1.8,0.));
#9630=CARTESIAN_POINT('',(3.8,-1.8,0.));
#9631=CARTESIAN_POINT('',(16.4,-1.8,0.));
#9632=CARTESIAN_POINT('',(16.4,-1.8,0.));
#9633=CARTESIAN_POINT('',(16.4,-3.2,0.));
#9634=CARTESIAN_POINT('',(16.4,-3.2,0.));
#9635=CARTESIAN_POINT('',(3.8,-3.2,0.));
#9636=CARTESIAN_POINT('',(3.8,-3.2,0.));
#9637=CARTESIAN_POINT('',(3.46875216140085,-3.00822493554786,0.));
#9638=CARTESIAN_POINT('',(0.,-1.,0.));
#9639=CARTESIAN_POINT('',(0.544110909138566,-1.31501157897496,0.));
#9640=CARTESIAN_POINT('Origin',(2.1,-2.,0.));
#9641=CARTESIAN_POINT('',(0.,-1.,0.));
#9642=CARTESIAN_POINT('Origin',(2.1,-2.,0.5));
#9643=CARTESIAN_POINT('Origin',(3.3,-2.,0.5));
#9644=CARTESIAN_POINT('Origin',(2.1,-2.,0.));
#9645=CARTESIAN_POINT('',(2.31345400686719,-0.313454006867188,0.));
#9646=CARTESIAN_POINT('',(3.78654599313281,-1.78654599313281,0.));
#9647=CARTESIAN_POINT('Origin',(2.1,-2.,0.));
#9648=CARTESIAN_POINT('',(0.544110909138566,-1.31501157897496,0.));
#9649=CARTESIAN_POINT('',(3.46875216140085,-3.00822493554786,0.));
#9650=CARTESIAN_POINT('Origin',(0.,-1.,0.));
#9651=CARTESIAN_POINT('',(3.8,-3.2,0.));
#9652=CARTESIAN_POINT('Origin',(3.8,-1.8,0.));
#9653=CARTESIAN_POINT('',(3.8,-1.8,0.));
#9654=CARTESIAN_POINT('Origin',(0.,-1.,0.));
#9655=CARTESIAN_POINT('Origin',(1.,1.,0.));
#9656=CARTESIAN_POINT('',(1.,1.,0.));
#9657=CARTESIAN_POINT('Origin',(3.8,-1.8,0.));
#9658=CARTESIAN_POINT('Origin',(16.4,-1.8,0.));
#9659=CARTESIAN_POINT('',(16.4,-1.8,0.));
#9660=CARTESIAN_POINT('Origin',(16.4,-3.2,0.));
#9661=CARTESIAN_POINT('',(16.4,-3.2,0.));
#9662=CARTESIAN_POINT('Origin',(3.8,-3.2,0.));
#19595=UNCERTAINTY_MEASURE_WITH_UNIT(LENGTH_MEASURE(0.001),#19619,
'DISTANCE_ACCURACY_VALUE',
'Maximum model space distance between geometric entities at asserted c
onnectivities');
#19605=UNCERTAINTY_MEASURE_WITH_UNIT(LENGTH_MEASURE(0.001),#19619,
'DISTANCE_ACCURACY_VALUE',
'Maximum model space distance between geometric entities at asserted c
onnectivities');
#19608=(
GEOMETRIC_REPRESENTATION_CONTEXT(3)
GLOBAL_UNCERTAINTY_ASSIGNED_CONTEXT((#19595))
GLOBAL_UNIT_ASSIGNED_CONTEXT((#19619,#19621,#19622))
REPRESENTATION_CONTEXT('','3D')
);
#19618=(
GEOMETRIC_REPRESENTATION_CONTEXT(3)
GLOBAL_UNCERTAINTY_ASSIGNED_CONTEXT((#19605))
GLOBAL_UNIT_ASSIGNED_CONTEXT((#19619,#19621,#19622))
REPRESENTATION_CONTEXT('','3D')
);
#19619=(
LENGTH_UNIT()
NAMED_UNIT(*)
SI_UNIT(.CENTI.,.METRE.)
);
#19621=(
NAMED_UNIT(*)
PLANE_ANGLE_UNIT()
SI_UNIT($,.RADIAN.)
);
#19622=(
NAMED_UNIT(*)
SI_UNIT($,.STERADIAN.)
SOLID_ANGLE_UNIT()
);
#19625=SHAPE_DEFINITION_REPRESENTATION(#19637,#19665);
#19637=PRODUCT_DEFINITION_SHAPE('',$,#19678);
#19665=SHAPE_REPRESENTATION('',(#7285),#19608);
#19675=PRODUCT_DEFINITION_CONTEXT('part definition',#19713,'design');
#19678=PRODUCT_DEFINITION('Moving jaw and handle',
'Moving jaw and handle',#19690,#19675);
#19690=PRODUCT_DEFINITION_FORMATION('',$,#19717);
#19713=APPLICATION_CONTEXT(
'Core Data for Automotive Mechanical Design Process');
#19714=PRODUCT_CONTEXT('part definition',#19713,'mechanical');
#19717=PRODUCT('Moving jaw and handle','Moving jaw and handle',$,(#19714));
#19728=PRESENTATION_STYLE_ASSIGNMENT((#19736));
#19736=SURFACE_STYLE_USAGE(.BOTH.,#19744);
#19744=SURFACE_SIDE_STYLE('',(#19752));
#19752=SURFACE_STYLE_FILL_AREA(#19760);
#19760=FILL_AREA_STYLE('Tool steel gray',(#19768));
#19768=FILL_AREA_STYLE_COLOUR('Tool steel gray',#19776);
#19776=COLOUR_RGB('Tool steel gray',0.607843137254902,0.643137254901961,
0.698039215686274);
ENDSEC;
END-ISO-10303-21;
